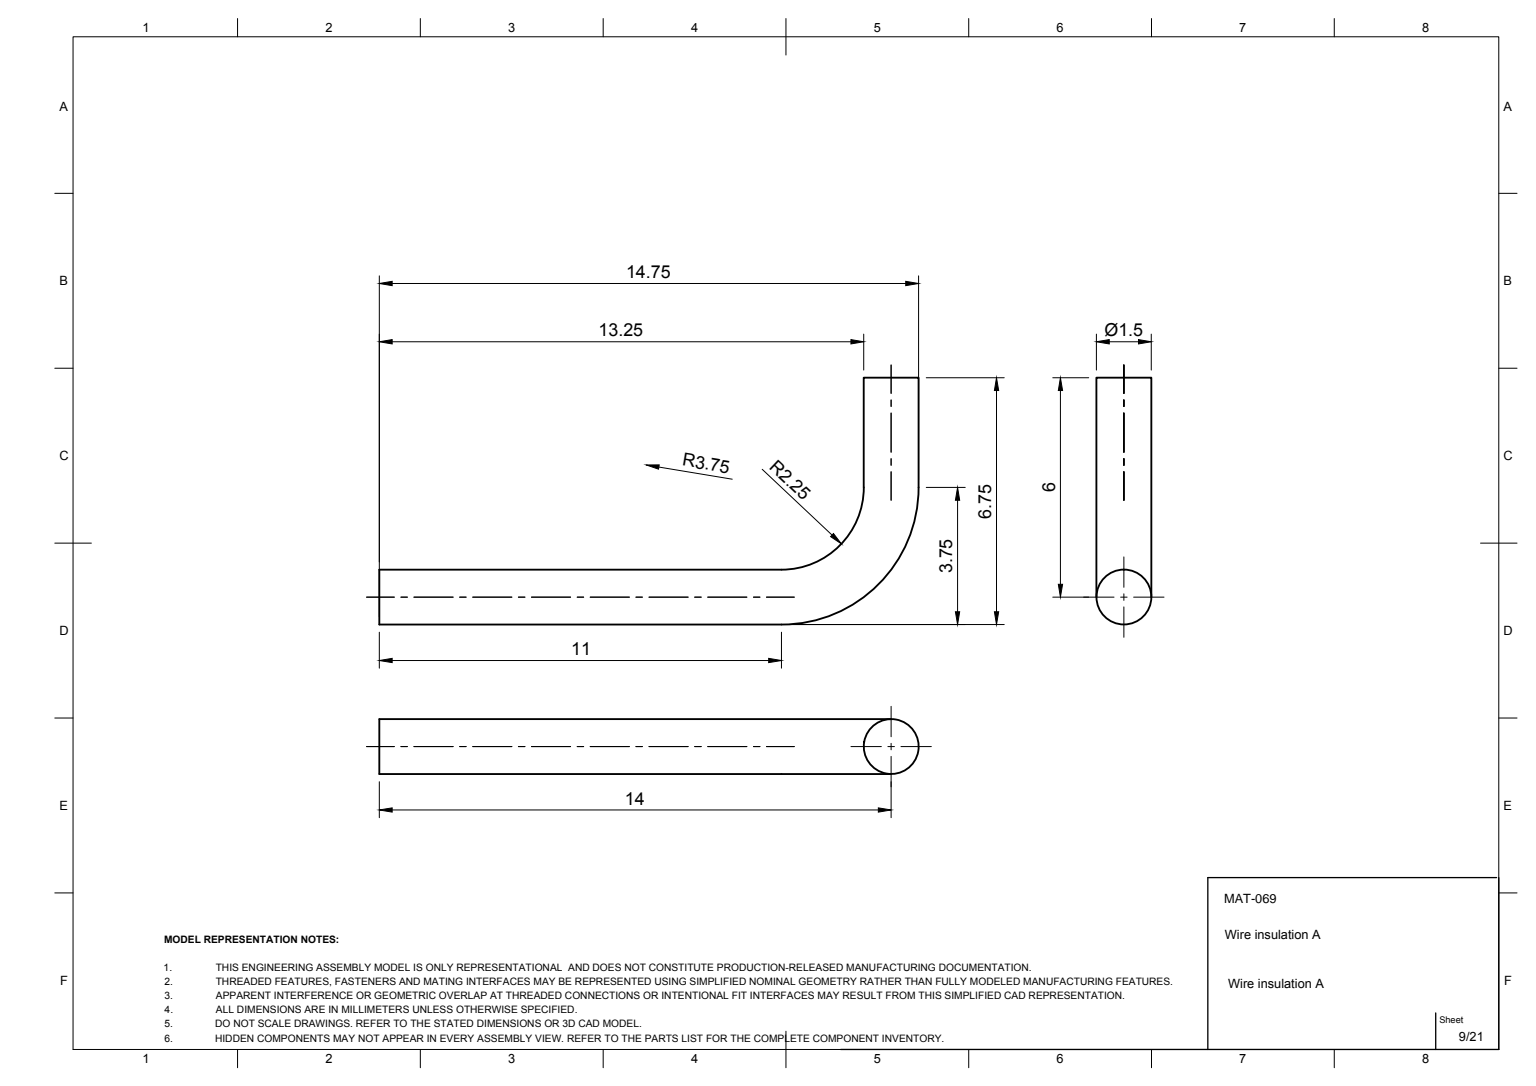
ISO-10303-21;
HEADER;
/* Generated by software containing ST-Developer
 * from STEP Tools, Inc. (www.steptools.com) 
 */

FILE_DESCRIPTION(
/* description */ ('CAx-IF Rec.Pracs.---Representation and Presentation of Product Manufa
cturing Information (PMI)---4.0---2014-10-13'),
/* implementation_level */ '2;1');

FILE_NAME(
/* name */ 'Wire insulation A.step',
/* time_stamp */ '2026-10-24T15:08:39-07:00',
/* author */ (''),
/* organization */ (''),
/* preprocessor_version */ 'ST-DEVELOPER v20.2',
/* originating_system */ 'Autodesk Translation Framework v15.17.0.0',
/* authorisation */ '');

FILE_SCHEMA (('AP242_MANAGED_MODEL_BASED_3D_ENGINEERING_MIM_LF { 1 0 10303 442 2 1 4 }'));
ENDSEC;

DATA;
#10=MECHANICAL_DESIGN_GEOMETRIC_PRESENTATION_REPRESENTATION('',(#826),#50081);
#773=TOROIDAL_SURFACE('',#10434,0.003,0.00075);
#786=SHAPE_REPRESENTATION_RELATIONSHIP('SRR','None',#50154,#806);
#806=ADVANCED_BREP_SHAPE_REPRESENTATION('',(#846),#50067);
#826=STYLED_ITEM('',(#50259),#846);
#846=MANIFOLD_SOLID_BREP('Body1',#9871);
#954=PLANE('',#10428);
#955=PLANE('',#10439);
#1261=FACE_OUTER_BOUND('',#1833,.T.);
#1262=FACE_OUTER_BOUND('',#1834,.T.);
#1263=FACE_OUTER_BOUND('',#1835,.T.);
#1264=FACE_OUTER_BOUND('',#1836,.T.);
#1265=FACE_OUTER_BOUND('',#1837,.T.);
#1833=EDGE_LOOP('',(#6998));
#1834=EDGE_LOOP('',(#6999,#7000,#7001,#7002,#7003));
#1835=EDGE_LOOP('',(#7004,#7005,#7006,#7007,#7008,#7009));
#1836=EDGE_LOOP('',(#7010,#7011,#7012,#7013,#7014));
#1837=EDGE_LOOP('',(#7015));
#2397=LINE('',#18084,#2975);
#2398=LINE('',#18095,#2976);
#2975=VECTOR('',#11841,0.00075);
#2976=VECTOR('',#11856,0.00075);
#3538=CIRCLE('',#10429,0.00075000000001);
#3539=CIRCLE('',#10431,0.00075000000001);
#3540=CIRCLE('',#10432,0.00075000000001);
#3541=CIRCLE('',#10433,0.00075000000001);
#3542=CIRCLE('',#10435,0.00225);
#3543=CIRCLE('',#10436,0.00075000000001);
#3544=CIRCLE('',#10437,0.00075000000001);
#4038=VERTEX_POINT('',#18078);
#4039=VERTEX_POINT('',#18081);
#4040=VERTEX_POINT('',#18083);
#4041=VERTEX_POINT('',#18085);
#4042=VERTEX_POINT('',#18089);
#4043=VERTEX_POINT('',#18091);
#5152=EDGE_CURVE('',#4038,#4038,#3538,.T.);
#5153=EDGE_CURVE('',#4039,#4039,#3539,.T.);
#5154=EDGE_CURVE('',#4039,#4040,#2397,.T.);
#5155=EDGE_CURVE('',#4040,#4041,#3540,.T.);
#5156=EDGE_CURVE('',#4041,#4040,#3541,.T.);
#5157=EDGE_CURVE('',#4041,#4042,#3542,.T.);
#5158=EDGE_CURVE('',#4042,#4043,#3543,.T.);
#5159=EDGE_CURVE('',#4043,#4042,#3544,.T.);
#5160=EDGE_CURVE('',#4043,#4038,#2398,.T.);
#6998=ORIENTED_EDGE('',*,*,#5152,.F.);
#6999=ORIENTED_EDGE('',*,*,#5153,.F.);
#7000=ORIENTED_EDGE('',*,*,#5154,.T.);
#7001=ORIENTED_EDGE('',*,*,#5155,.T.);
#7002=ORIENTED_EDGE('',*,*,#5156,.T.);
#7003=ORIENTED_EDGE('',*,*,#5154,.F.);
#7004=ORIENTED_EDGE('',*,*,#5156,.F.);
#7005=ORIENTED_EDGE('',*,*,#5157,.T.);
#7006=ORIENTED_EDGE('',*,*,#5158,.T.);
#7007=ORIENTED_EDGE('',*,*,#5159,.T.);
#7008=ORIENTED_EDGE('',*,*,#5157,.F.);
#7009=ORIENTED_EDGE('',*,*,#5155,.F.);
#7010=ORIENTED_EDGE('',*,*,#5159,.F.);
#7011=ORIENTED_EDGE('',*,*,#5160,.T.);
#7012=ORIENTED_EDGE('',*,*,#5152,.T.);
#7013=ORIENTED_EDGE('',*,*,#5160,.F.);
#7014=ORIENTED_EDGE('',*,*,#5158,.F.);
#7015=ORIENTED_EDGE('',*,*,#5153,.T.);
#9180=CYLINDRICAL_SURFACE('',#10430,0.00075);
#9181=CYLINDRICAL_SURFACE('',#10438,0.00075);
#9483=ADVANCED_FACE('',(#1261),#954,.F.);
#9484=ADVANCED_FACE('',(#1262),#9180,.T.);
#9485=ADVANCED_FACE('',(#1263),#773,.T.);
#9486=ADVANCED_FACE('',(#1264),#9181,.T.);
#9487=ADVANCED_FACE('',(#1265),#955,.T.);
#9871=CLOSED_SHELL('',(#9483,#9484,#9485,#9486,#9487));
#10427=AXIS2_PLACEMENT_3D('',#18076,#11831,#11832);
#10428=AXIS2_PLACEMENT_3D('',#18077,#11833,#11834);
#10429=AXIS2_PLACEMENT_3D('',#18079,#11835,#11836);
#10430=AXIS2_PLACEMENT_3D('',#18080,#11837,#11838);
#10431=AXIS2_PLACEMENT_3D('',#18082,#11839,#11840);
#10432=AXIS2_PLACEMENT_3D('',#18086,#11842,#11843);
#10433=AXIS2_PLACEMENT_3D('',#18087,#11844,#11845);
#10434=AXIS2_PLACEMENT_3D('',#18088,#11846,#11847);
#10435=AXIS2_PLACEMENT_3D('',#18090,#11848,#11849);
#10436=AXIS2_PLACEMENT_3D('',#18092,#11850,#11851);
#10437=AXIS2_PLACEMENT_3D('',#18093,#11852,#11853);
#10438=AXIS2_PLACEMENT_3D('',#18094,#11854,#11855);
#10439=AXIS2_PLACEMENT_3D('',#18096,#11857,#11858);
#11831=DIRECTION('axis',(0.,0.,1.));
#11832=DIRECTION('refdir',(1.,0.,0.));
#11833=DIRECTION('center_axis',(0.984807753012209,-0.173648177666927,-6.9026791896102E-15));
#11834=DIRECTION('ref_axis',(6.74488507274914E-15,-1.49880108324396E-15,
1.));
#11835=DIRECTION('center_axis',(0.984807753012209,-0.173648177666927,-6.9026791896102E-15));
#11836=DIRECTION('ref_axis',(-0.173648177666927,-0.984807753012209,-1.41609297436625E-15));
#11837=DIRECTION('center_axis',(-6.74488507274914E-15,1.49880108324396E-15,
-1.));
#11838=DIRECTION('ref_axis',(-0.173648177666927,-0.984807753012209,-3.04793925546002E-16));
#11839=DIRECTION('center_axis',(1.31243041282465E-11,-2.31385942497016E-12,
-1.));
#11840=DIRECTION('ref_axis',(-0.173648177666927,-0.984807753012209,-3.04793925546223E-16));
#11841=DIRECTION('',(6.74488507274914E-15,-1.49880108324396E-15,1.));
#11842=DIRECTION('center_axis',(1.31243041282465E-11,-2.31385942497016E-12,
-1.));
#11843=DIRECTION('ref_axis',(-0.173648177666927,-0.984807753012209,-3.04793925546223E-16));
#11844=DIRECTION('center_axis',(1.31243041282465E-11,-2.31385942497016E-12,
-1.));
#11845=DIRECTION('ref_axis',(-0.173648177666927,-0.984807753012209,-3.04793925546223E-16));
#11846=DIRECTION('center_axis',(0.173648177666927,0.984807753012209,1.41609297436625E-15));
#11847=DIRECTION('ref_axis',(-6.47630097698008E-15,1.85037170770859E-15,
-1.));
#11848=DIRECTION('center_axis',(-0.173648177666927,-0.984807753012209,-1.41609297436625E-15));
#11849=DIRECTION('ref_axis',(-6.31282311555423E-15,2.55105953078819E-15,
-1.));
#11850=DIRECTION('center_axis',(0.984807753012209,-0.173648177666927,-6.9026791896102E-15));
#11851=DIRECTION('ref_axis',(-0.173648177666927,-0.984807753012209,-1.41609297436625E-15));
#11852=DIRECTION('center_axis',(0.984807753012209,-0.173648177666927,-6.9026791896102E-15));
#11853=DIRECTION('ref_axis',(-0.173648177666927,-0.984807753012209,-1.41609297436625E-15));
#11854=DIRECTION('center_axis',(0.984807753012209,-0.173648177666927,-6.9026791896102E-15));
#11855=DIRECTION('ref_axis',(-0.173648177666927,-0.984807753012209,-1.41609297436625E-15));
#11856=DIRECTION('',(-0.984807753012209,0.173648177666927,6.9026791896102E-15));
#11857=DIRECTION('center_axis',(-6.46591174117934E-15,1.44961055799008E-15,
-1.));
#11858=DIRECTION('ref_axis',(-0.173648177666927,-0.984807753012209,-3.04793925546006E-16));
#18076=CARTESIAN_POINT('',(0.,0.,0.));
#18077=CARTESIAN_POINT('Origin',(-0.0200268362756705,-0.033370488273017,
0.0038241467581455));
#18078=CARTESIAN_POINT('',(-0.0198966001424301,-0.0326318824582561,0.0038241467581455));
#18079=CARTESIAN_POINT('Origin',(-0.0200268362756803,-0.0333704882730153,
0.0038241467581555));
#18080=CARTESIAN_POINT('Origin',(-0.00623952773349959,-0.035801562760354,
0.000824146758145402));
#18081=CARTESIAN_POINT('',(-0.00610929160024941,-0.0350629569455948,-0.00217585328655807));
#18082=CARTESIAN_POINT('Origin',(-0.00623952773350945,-0.0358015627603522,
-0.00217585328654807));
#18083=CARTESIAN_POINT('',(-0.00610929160024939,-0.0350629569455948,0.000824146758165404));
#18084=CARTESIAN_POINT('',(-0.00610929160024939,-0.0350629569455948,0.000824146758145402));
#18085=CARTESIAN_POINT('',(-0.00697813354827845,-0.0356713266271003,0.000824146758145408));
#18086=CARTESIAN_POINT('Origin',(-0.00623952773350944,-0.0358015627603522,
0.000824146758155403));
#18087=CARTESIAN_POINT('Origin',(-0.00623952773350944,-0.0358015627603522,
0.000824146758155403));
#18088=CARTESIAN_POINT('Origin',(-0.00919395099253621,-0.0352806182273532,
0.000824146758145423));
#18089=CARTESIAN_POINT('',(-0.00919395099254606,-0.0352806182273515,0.00307414675814542));
#18090=CARTESIAN_POINT('Origin',(-0.00919395099253621,-0.0352806182273532,
0.000824146758145423));
#18091=CARTESIAN_POINT('',(-0.00906371485929584,-0.0345420124125923,0.00382414675814543));
#18092=CARTESIAN_POINT('Origin',(-0.00919395099254604,-0.0352806182273514,
0.00382414675815542));
#18093=CARTESIAN_POINT('Origin',(-0.00919395099254604,-0.0352806182273514,
0.00382414675815542));
#18094=CARTESIAN_POINT('Origin',(-0.0239660672877193,-0.0326758955623493,
0.00382414675814553));
#18095=CARTESIAN_POINT('',(-0.0238358311544691,-0.0319372897475901,0.00382414675814553));
#18096=CARTESIAN_POINT('Origin',(-0.00623952773349961,-0.035801562760354,
-0.00217585328655807));
#50045=UNCERTAINTY_MEASURE_WITH_UNIT(LENGTH_MEASURE(1.E-5),#50082,
'DISTANCE_ACCURACY_VALUE',
'Maximum model space distance between geometric entities at asserted c
onnectivities');
#50059=UNCERTAINTY_MEASURE_WITH_UNIT(LENGTH_MEASURE(1.E-5),#50082,
'DISTANCE_ACCURACY_VALUE',
'Maximum model space distance between geometric entities at asserted c
onnectivities');
#50067=(
GEOMETRIC_REPRESENTATION_CONTEXT(3)
GLOBAL_UNCERTAINTY_ASSIGNED_CONTEXT((#50045))
GLOBAL_UNIT_ASSIGNED_CONTEXT((#50082,#50083,#50084))
REPRESENTATION_CONTEXT('','3D')
);
#50081=(
GEOMETRIC_REPRESENTATION_CONTEXT(3)
GLOBAL_UNCERTAINTY_ASSIGNED_CONTEXT((#50059))
GLOBAL_UNIT_ASSIGNED_CONTEXT((#50082,#50083,#50084))
REPRESENTATION_CONTEXT('','3D')
);
#50082=(
LENGTH_UNIT()
NAMED_UNIT(*)
SI_UNIT($,.METRE.)
);
#50083=(
NAMED_UNIT(*)
PLANE_ANGLE_UNIT()
SI_UNIT($,.RADIAN.)
);
#50084=(
NAMED_UNIT(*)
SI_UNIT($,.STERADIAN.)
SOLID_ANGLE_UNIT()
);
#50092=SHAPE_DEFINITION_REPRESENTATION(#50113,#50154);
#50113=PRODUCT_DEFINITION_SHAPE('',$,#50176);
#50154=SHAPE_REPRESENTATION('',(#10427),#50067);
#50168=PRODUCT_DEFINITION_CONTEXT('part definition',#50233,'design');
#50176=PRODUCT_DEFINITION('Wire insulation A','Wire insulation A',#50197,
#50168);
#50197=PRODUCT_DEFINITION_FORMATION('',$,#50242);
#50233=APPLICATION_CONTEXT('Managed model based 3d engineering');
#50234=PRODUCT_CONTEXT('part definition',#50233,'mechanical');
#50242=PRODUCT('Wire insulation A','Wire insulation A',
'LEGAL AND USAGE DISCLAIMER: this Data/Model is provided \X2\201C\X0\A
S IS\X2\201D\X0\ for informational and representational only. It is a 
geometric approximation and is NOT engineered, certified, or guarantee
d for dimensional accuracy, exact tolerances, or production-level prec
ision. Vendor disclaims all implied warranties including fitness for a
 particular purpose. DO NOT USE FOR DIRECT PHYSICAL MANUFACTURING, AUT
OMATED PRODUCTION, OR SAFETY-CRITICAL SYSTEMS without independent engi
neering verification and resolution of any design discrepancies.',(#50234));
#50259=PRESENTATION_STYLE_ASSIGNMENT((#50266));
#50266=SURFACE_STYLE_USAGE(.BOTH.,#50273);
#50273=SURFACE_SIDE_STYLE('',(#50280));
#50280=SURFACE_STYLE_FILL_AREA(#50287);
#50287=FILL_AREA_STYLE('Opaque(246,246,243)',(#50294));
#50294=FILL_AREA_STYLE_COLOUR('Opaque(246,246,243)',#50301);
#50301=COLOUR_RGB('Opaque(246,246,243)',0.964705882352941,0.964705882352941,
0.952941176470588);
ENDSEC;
END-ISO-10303-21;
